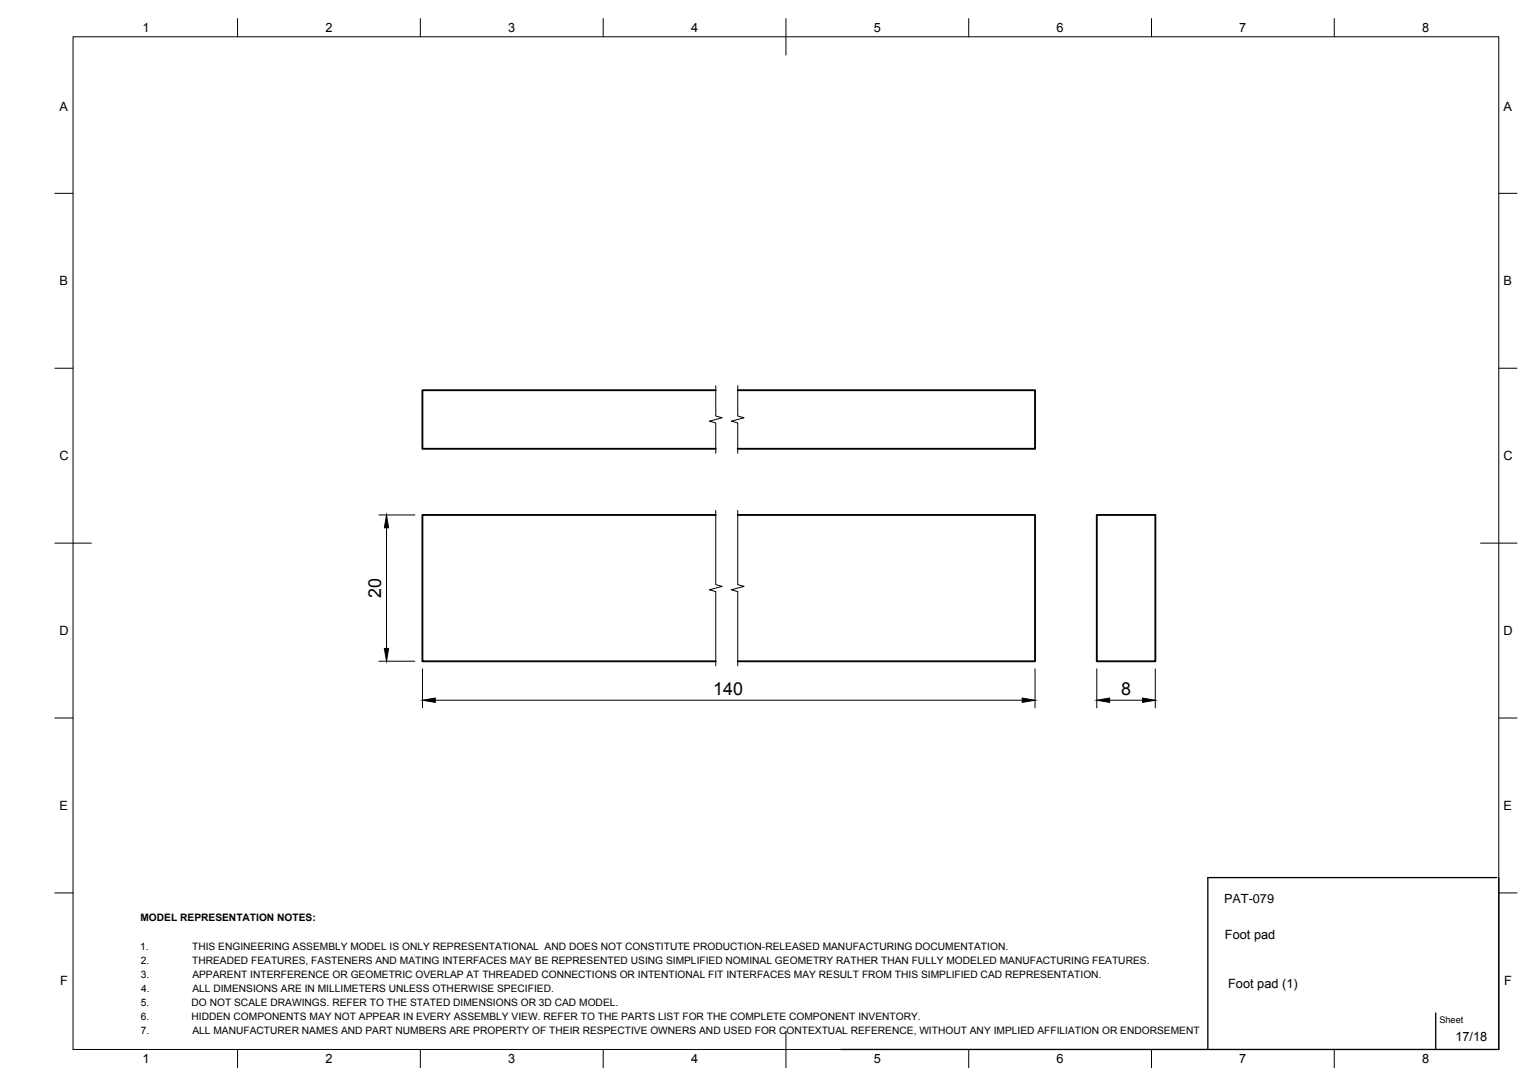
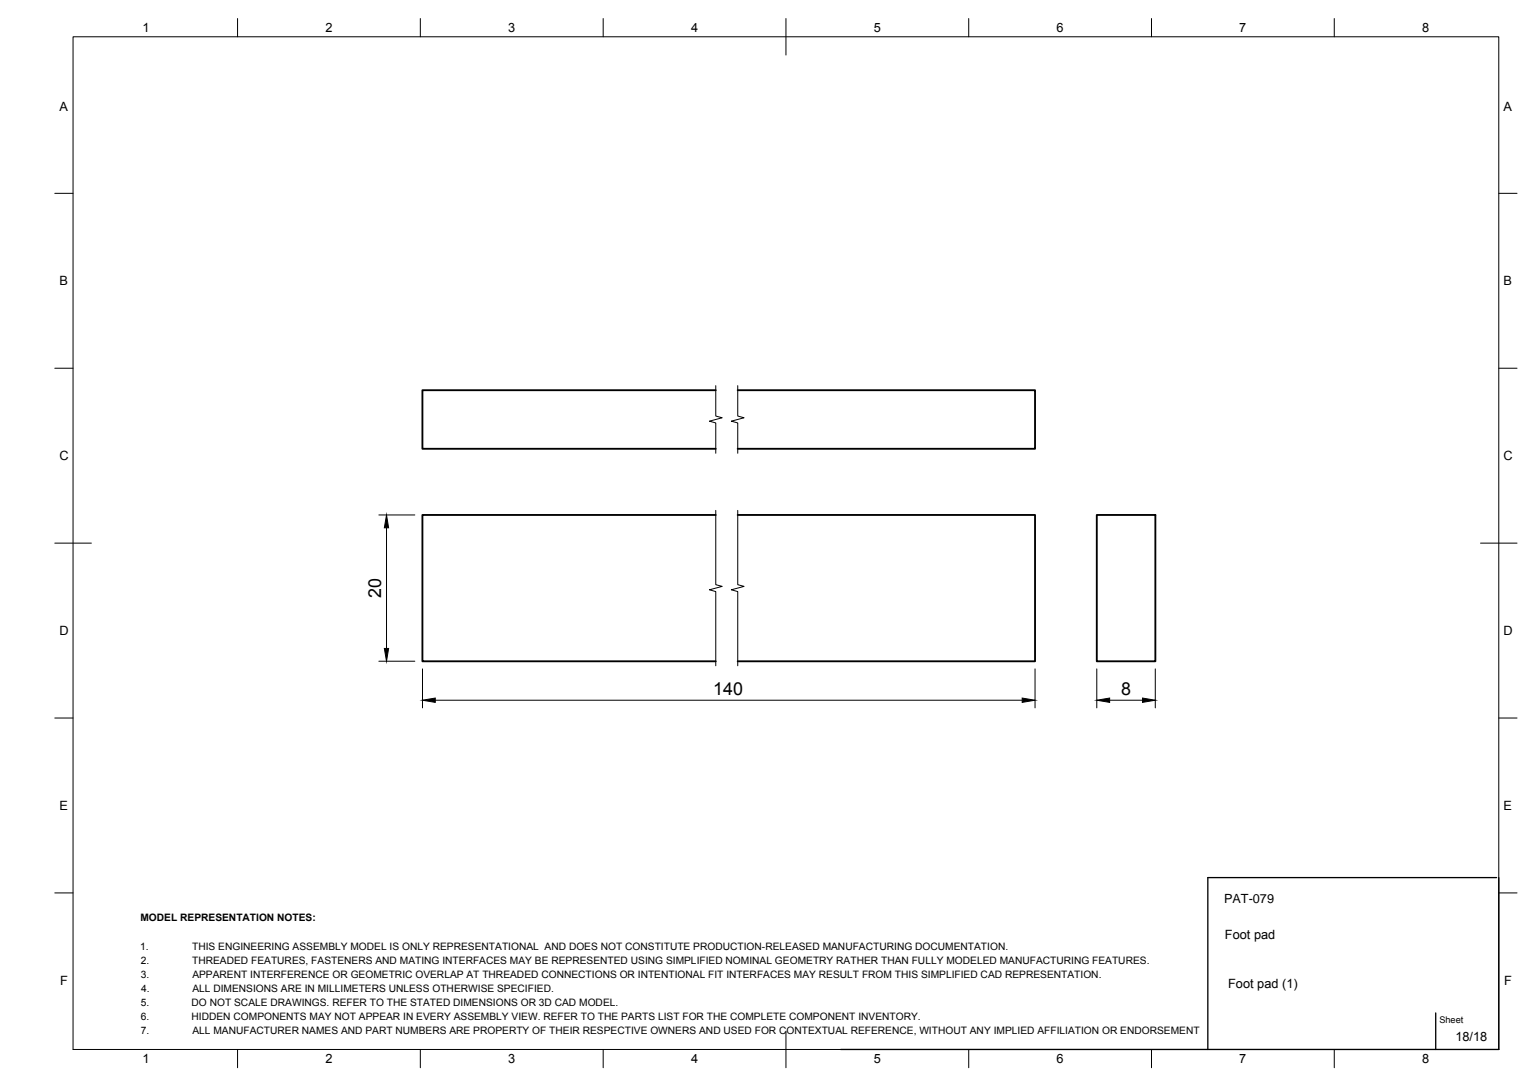
ISO-10303-21;
HEADER;
/* Generated by software containing ST-Developer
 * from STEP Tools, Inc. (www.steptools.com) 
 */

FILE_DESCRIPTION(
/* description */ ('Pipe clamp stand with threaded column'),
/* implementation_level */ '2;1');

FILE_NAME(
/* name */ 'Foot pad (1).step',
/* time_stamp */ '2026-10-27T10:55:48-07:00',
/* author */ (''),
/* organization */ (''),
/* preprocessor_version */ 'ST-DEVELOPER v20.2',
/* originating_system */ 'Autodesk Translation Framework v15.17.0.0',
/* authorisation */ '');

FILE_SCHEMA (('AUTOMOTIVE_DESIGN { 1 0 10303 214 3 1 1 }'));
ENDSEC;

DATA;
#10=MECHANICAL_DESIGN_GEOMETRIC_PRESENTATION_REPRESENTATION('',(#762),#34433);
#710=SHAPE_REPRESENTATION_RELATIONSHIP('SRR','None',#34552,#732);
#732=ADVANCED_BREP_SHAPE_REPRESENTATION('',(#792),#34420);
#762=STYLED_ITEM('',(#34736),#792);
#792=MANIFOLD_SOLID_BREP('Body1',#8789);
#973=PLANE('',#9503);
#974=PLANE('',#9504);
#975=PLANE('',#9505);
#976=PLANE('',#9506);
#977=PLANE('',#9507);
#978=PLANE('',#9508);
#1396=FACE_OUTER_BOUND('',#1926,.T.);
#1397=FACE_OUTER_BOUND('',#1927,.T.);
#1398=FACE_OUTER_BOUND('',#1928,.T.);
#1399=FACE_OUTER_BOUND('',#1929,.T.);
#1400=FACE_OUTER_BOUND('',#1930,.T.);
#1401=FACE_OUTER_BOUND('',#1931,.T.);
#1926=EDGE_LOOP('',(#7355,#7356,#7357,#7358));
#1927=EDGE_LOOP('',(#7359,#7360,#7361,#7362));
#1928=EDGE_LOOP('',(#7363,#7364,#7365,#7366));
#1929=EDGE_LOOP('',(#7367,#7368,#7369,#7370));
#1930=EDGE_LOOP('',(#7371,#7372,#7373,#7374));
#1931=EDGE_LOOP('',(#7375,#7376,#7377,#7378));
#2519=LINE('',#28655,#3136);
#2520=LINE('',#28657,#3137);
#2521=LINE('',#28659,#3138);
#2522=LINE('',#28660,#3139);
#2523=LINE('',#28663,#3140);
#2524=LINE('',#28665,#3141);
#2525=LINE('',#28666,#3142);
#2526=LINE('',#28669,#3143);
#2527=LINE('',#28671,#3144);
#2528=LINE('',#28672,#3145);
#2529=LINE('',#28674,#3146);
#2530=LINE('',#28675,#3147);
#3136=VECTOR('',#11090,1.);
#3137=VECTOR('',#11091,1.);
#3138=VECTOR('',#11092,1.);
#3139=VECTOR('',#11093,1.);
#3140=VECTOR('',#11096,1.);
#3141=VECTOR('',#11097,1.);
#3142=VECTOR('',#11098,1.);
#3143=VECTOR('',#11101,1.);
#3144=VECTOR('',#11102,1.);
#3145=VECTOR('',#11103,1.);
#3146=VECTOR('',#11106,1.);
#3147=VECTOR('',#11107,1.);
#4058=VERTEX_POINT('',#28653);
#4059=VERTEX_POINT('',#28654);
#4060=VERTEX_POINT('',#28656);
#4061=VERTEX_POINT('',#28658);
#4062=VERTEX_POINT('',#28662);
#4063=VERTEX_POINT('',#28664);
#4064=VERTEX_POINT('',#28668);
#4065=VERTEX_POINT('',#28670);
#5191=EDGE_CURVE('',#4058,#4059,#2519,.T.);
#5192=EDGE_CURVE('',#4059,#4060,#2520,.T.);
#5193=EDGE_CURVE('',#4061,#4060,#2521,.T.);
#5194=EDGE_CURVE('',#4058,#4061,#2522,.T.);
#5195=EDGE_CURVE('',#4062,#4058,#2523,.T.);
#5196=EDGE_CURVE('',#4063,#4061,#2524,.T.);
#5197=EDGE_CURVE('',#4062,#4063,#2525,.T.);
#5198=EDGE_CURVE('',#4064,#4062,#2526,.T.);
#5199=EDGE_CURVE('',#4065,#4063,#2527,.T.);
#5200=EDGE_CURVE('',#4064,#4065,#2528,.T.);
#5201=EDGE_CURVE('',#4059,#4064,#2529,.T.);
#5202=EDGE_CURVE('',#4060,#4065,#2530,.T.);
#7355=ORIENTED_EDGE('',*,*,#5191,.T.);
#7356=ORIENTED_EDGE('',*,*,#5192,.T.);
#7357=ORIENTED_EDGE('',*,*,#5193,.F.);
#7358=ORIENTED_EDGE('',*,*,#5194,.F.);
#7359=ORIENTED_EDGE('',*,*,#5195,.T.);
#7360=ORIENTED_EDGE('',*,*,#5194,.T.);
#7361=ORIENTED_EDGE('',*,*,#5196,.F.);
#7362=ORIENTED_EDGE('',*,*,#5197,.F.);
#7363=ORIENTED_EDGE('',*,*,#5198,.T.);
#7364=ORIENTED_EDGE('',*,*,#5197,.T.);
#7365=ORIENTED_EDGE('',*,*,#5199,.F.);
#7366=ORIENTED_EDGE('',*,*,#5200,.F.);
#7367=ORIENTED_EDGE('',*,*,#5201,.T.);
#7368=ORIENTED_EDGE('',*,*,#5200,.T.);
#7369=ORIENTED_EDGE('',*,*,#5202,.F.);
#7370=ORIENTED_EDGE('',*,*,#5192,.F.);
#7371=ORIENTED_EDGE('',*,*,#5202,.T.);
#7372=ORIENTED_EDGE('',*,*,#5199,.T.);
#7373=ORIENTED_EDGE('',*,*,#5196,.T.);
#7374=ORIENTED_EDGE('',*,*,#5193,.T.);
#7375=ORIENTED_EDGE('',*,*,#5201,.F.);
#7376=ORIENTED_EDGE('',*,*,#5191,.F.);
#7377=ORIENTED_EDGE('',*,*,#5195,.F.);
#7378=ORIENTED_EDGE('',*,*,#5198,.F.);
#8633=ADVANCED_FACE('',(#1396),#973,.T.);
#8634=ADVANCED_FACE('',(#1397),#974,.T.);
#8635=ADVANCED_FACE('',(#1398),#975,.T.);
#8636=ADVANCED_FACE('',(#1399),#976,.T.);
#8637=ADVANCED_FACE('',(#1400),#977,.T.);
#8638=ADVANCED_FACE('',(#1401),#978,.F.);
#8789=CLOSED_SHELL('',(#8633,#8634,#8635,#8636,#8637,#8638));
#9502=AXIS2_PLACEMENT_3D('',#28651,#11086,#11087);
#9503=AXIS2_PLACEMENT_3D('',#28652,#11088,#11089);
#9504=AXIS2_PLACEMENT_3D('',#28661,#11094,#11095);
#9505=AXIS2_PLACEMENT_3D('',#28667,#11099,#11100);
#9506=AXIS2_PLACEMENT_3D('',#28673,#11104,#11105);
#9507=AXIS2_PLACEMENT_3D('',#28676,#11108,#11109);
#9508=AXIS2_PLACEMENT_3D('',#28677,#11110,#11111);
#11086=DIRECTION('axis',(0.,0.,1.));
#11087=DIRECTION('refdir',(1.,0.,0.));
#11088=DIRECTION('center_axis',(0.,1.,0.));
#11089=DIRECTION('ref_axis',(-1.,0.,0.));
#11090=DIRECTION('',(-1.,0.,0.));
#11091=DIRECTION('',(0.,0.,1.));
#11092=DIRECTION('',(-1.,0.,0.));
#11093=DIRECTION('',(0.,0.,1.));
#11094=DIRECTION('center_axis',(1.,0.,0.));
#11095=DIRECTION('ref_axis',(0.,1.,0.));
#11096=DIRECTION('',(0.,1.,0.));
#11097=DIRECTION('',(0.,1.,0.));
#11098=DIRECTION('',(0.,0.,1.));
#11099=DIRECTION('center_axis',(0.,-1.,0.));
#11100=DIRECTION('ref_axis',(1.,0.,0.));
#11101=DIRECTION('',(1.,0.,0.));
#11102=DIRECTION('',(1.,0.,0.));
#11103=DIRECTION('',(0.,0.,1.));
#11104=DIRECTION('center_axis',(-1.,0.,0.));
#11105=DIRECTION('ref_axis',(0.,-1.,0.));
#11106=DIRECTION('',(0.,-1.,0.));
#11107=DIRECTION('',(0.,-1.,0.));
#11108=DIRECTION('center_axis',(0.,0.,1.));
#11109=DIRECTION('ref_axis',(1.,0.,0.));
#11110=DIRECTION('center_axis',(0.,0.,1.));
#11111=DIRECTION('ref_axis',(1.,0.,0.));
#28651=CARTESIAN_POINT('',(0.,0.,0.));
#28652=CARTESIAN_POINT('Origin',(6.5,7.,-0.8));
#28653=CARTESIAN_POINT('',(6.5,7.,-0.8));
#28654=CARTESIAN_POINT('',(4.5,7.,-0.8));
#28655=CARTESIAN_POINT('',(6.5,7.,-0.8));
#28656=CARTESIAN_POINT('',(4.5,7.,0.));
#28657=CARTESIAN_POINT('',(4.5,7.,-0.8));
#28658=CARTESIAN_POINT('',(6.5,7.,0.));
#28659=CARTESIAN_POINT('',(6.5,7.,0.));
#28660=CARTESIAN_POINT('',(6.5,7.,-0.8));
#28661=CARTESIAN_POINT('Origin',(6.5,-7.,-0.8));
#28662=CARTESIAN_POINT('',(6.5,-7.,-0.8));
#28663=CARTESIAN_POINT('',(6.5,-7.,-0.8));
#28664=CARTESIAN_POINT('',(6.5,-7.,0.));
#28665=CARTESIAN_POINT('',(6.5,-7.,0.));
#28666=CARTESIAN_POINT('',(6.5,-7.,-0.8));
#28667=CARTESIAN_POINT('Origin',(4.5,-7.,-0.8));
#28668=CARTESIAN_POINT('',(4.5,-7.,-0.8));
#28669=CARTESIAN_POINT('',(4.5,-7.,-0.8));
#28670=CARTESIAN_POINT('',(4.5,-7.,0.));
#28671=CARTESIAN_POINT('',(4.5,-7.,0.));
#28672=CARTESIAN_POINT('',(4.5,-7.,-0.8));
#28673=CARTESIAN_POINT('Origin',(4.5,7.,-0.8));
#28674=CARTESIAN_POINT('',(4.5,7.,-0.8));
#28675=CARTESIAN_POINT('',(4.5,7.,0.));
#28676=CARTESIAN_POINT('Origin',(5.5,0.,0.));
#28677=CARTESIAN_POINT('Origin',(5.5,0.,-0.8));
#34391=UNCERTAINTY_MEASURE_WITH_UNIT(LENGTH_MEASURE(0.001),#34434,
'DISTANCE_ACCURACY_VALUE',
'Maximum model space distance between geometric entities at asserted c
onnectivities');
#34404=UNCERTAINTY_MEASURE_WITH_UNIT(LENGTH_MEASURE(0.001),#34434,
'DISTANCE_ACCURACY_VALUE',
'Maximum model space distance between geometric entities at asserted c
onnectivities');
#34420=(
GEOMETRIC_REPRESENTATION_CONTEXT(3)
GLOBAL_UNCERTAINTY_ASSIGNED_CONTEXT((#34391))
GLOBAL_UNIT_ASSIGNED_CONTEXT((#34434,#34436,#34437))
REPRESENTATION_CONTEXT('','3D')
);
#34433=(
GEOMETRIC_REPRESENTATION_CONTEXT(3)
GLOBAL_UNCERTAINTY_ASSIGNED_CONTEXT((#34404))
GLOBAL_UNIT_ASSIGNED_CONTEXT((#34434,#34436,#34437))
REPRESENTATION_CONTEXT('','3D')
);
#34434=(
LENGTH_UNIT()
NAMED_UNIT(*)
SI_UNIT(.CENTI.,.METRE.)
);
#34436=(
NAMED_UNIT(*)
PLANE_ANGLE_UNIT()
SI_UNIT($,.RADIAN.)
);
#34437=(
NAMED_UNIT(*)
SI_UNIT($,.STERADIAN.)
SOLID_ANGLE_UNIT()
);
#34453=SHAPE_DEFINITION_REPRESENTATION(#34481,#34552);
#34481=PRODUCT_DEFINITION_SHAPE('',$,#34581);
#34552=SHAPE_REPRESENTATION('',(#9502),#34420);
#34565=PRODUCT_DEFINITION_CONTEXT('part definition',#34651,'design');
#34581=PRODUCT_DEFINITION('Foot pad (1)','Foot pad (1)',#34609,#34565);
#34609=PRODUCT_DEFINITION_FORMATION('',$,#34668);
#34651=APPLICATION_CONTEXT(
'Core Data for Automotive Mechanical Design Process');
#34652=PRODUCT_CONTEXT('part definition',#34651,'mechanical');
#34668=PRODUCT('Foot pad (1)','Foot pad (1)','Foot pad (1)',(#34652));
#34730=COLOUR_RGB('Sky Blue',0.24,0.69,0.87);
#34731=FILL_AREA_STYLE_COLOUR('',#34730);
#34732=FILL_AREA_STYLE('',(#34731));
#34733=SURFACE_STYLE_FILL_AREA(#34732);
#34734=SURFACE_SIDE_STYLE('',(#34733));
#34735=SURFACE_STYLE_USAGE(.BOTH.,#34734);
#34736=PRESENTATION_STYLE_ASSIGNMENT((#34735));
ENDSEC;
END-ISO-10303-21;
